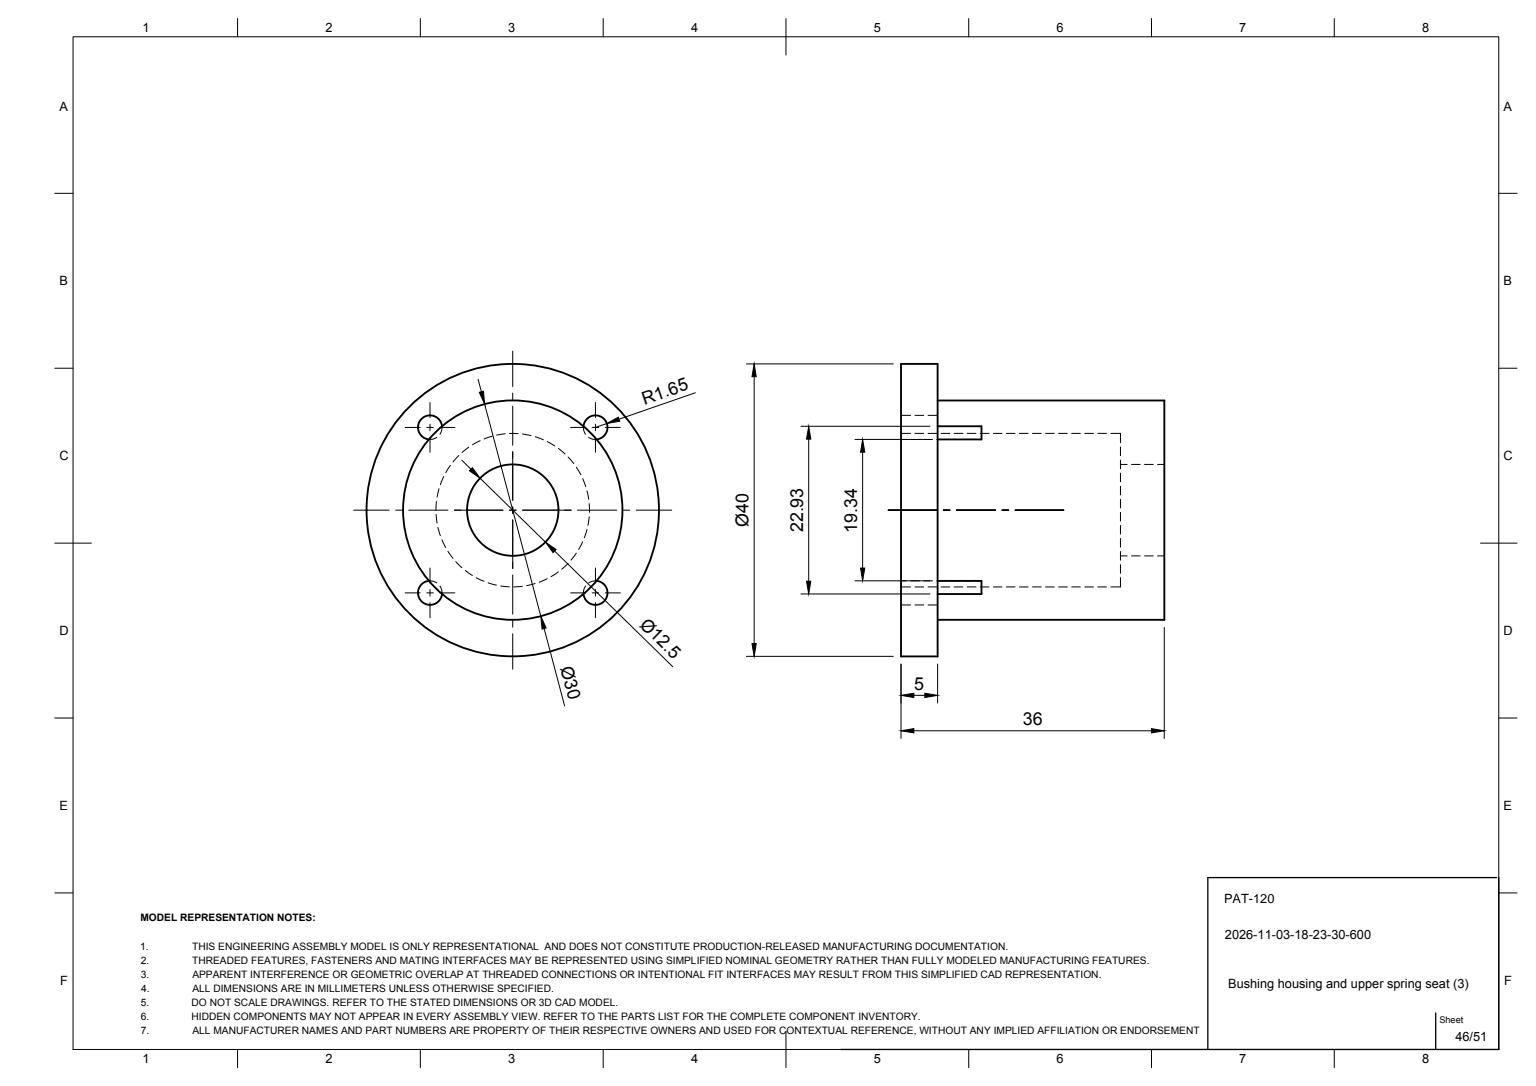
ISO-10303-21;
HEADER;
/* Generated by software containing ST-Developer
 * from STEP Tools, Inc. (www.steptools.com) 
 */

FILE_DESCRIPTION(
/* description */ ('Vibration shaker table dummy'),
/* implementation_level */ '2;1');

FILE_NAME(
/* name */ 'Bushing housing and upper spring seat (3).step',
/* time_stamp */ '2026-10-27T10:55:14-07:00',
/* author */ (''),
/* organization */ (''),
/* preprocessor_version */ 'ST-DEVELOPER v20.2',
/* originating_system */ 'Autodesk Translation Framework v15.17.0.0',
/* authorisation */ '');

FILE_SCHEMA (('AUTOMOTIVE_DESIGN { 1 0 10303 214 3 1 1 }'));
ENDSEC;

DATA;
#10=MECHANICAL_DESIGN_GEOMETRIC_PRESENTATION_REPRESENTATION('',(#727),#22394);
#635=SHAPE_REPRESENTATION_RELATIONSHIP('SRR','None',#22682,#681);
#681=ADVANCED_BREP_SHAPE_REPRESENTATION('',(#771),#22388);
#727=STYLED_ITEM('',(#22961),#771);
#771=MANIFOLD_SOLID_BREP('Body1',#9247);
#1031=FACE_BOUND('',#2537,.T.);
#1032=FACE_BOUND('',#2539,.T.);
#1033=FACE_BOUND('',#2543,.T.);
#1034=FACE_BOUND('',#2544,.T.);
#1035=FACE_BOUND('',#2545,.T.);
#1036=FACE_BOUND('',#2546,.T.);
#1037=FACE_BOUND('',#2547,.T.);
#1038=FACE_BOUND('',#2549,.T.);
#1302=PLANE('',#10665);
#1303=PLANE('',#10672);
#1304=PLANE('',#10679);
#1305=PLANE('',#10686);
#1306=PLANE('',#10703);
#1307=PLANE('',#10705);
#1308=PLANE('',#10711);
#1309=PLANE('',#10712);
#1772=FACE_OUTER_BOUND('',#2526,.T.);
#1773=FACE_OUTER_BOUND('',#2527,.T.);
#1774=FACE_OUTER_BOUND('',#2528,.T.);
#1775=FACE_OUTER_BOUND('',#2529,.T.);
#1776=FACE_OUTER_BOUND('',#2530,.T.);
#1777=FACE_OUTER_BOUND('',#2531,.T.);
#1778=FACE_OUTER_BOUND('',#2532,.T.);
#1779=FACE_OUTER_BOUND('',#2533,.T.);
#1780=FACE_OUTER_BOUND('',#2534,.T.);
#1781=FACE_OUTER_BOUND('',#2535,.T.);
#1782=FACE_OUTER_BOUND('',#2536,.T.);
#1783=FACE_OUTER_BOUND('',#2538,.T.);
#1784=FACE_OUTER_BOUND('',#2540,.T.);
#1785=FACE_OUTER_BOUND('',#2541,.T.);
#1786=FACE_OUTER_BOUND('',#2542,.T.);
#1787=FACE_OUTER_BOUND('',#2548,.T.);
#2526=EDGE_LOOP('',(#8214,#8215));
#2527=EDGE_LOOP('',(#8216,#8217,#8218,#8219,#8220,#8221,#8222,#8223));
#2528=EDGE_LOOP('',(#8224,#8225));
#2529=EDGE_LOOP('',(#8226,#8227,#8228,#8229,#8230,#8231,#8232,#8233));
#2530=EDGE_LOOP('',(#8234,#8235,#8236));
#2531=EDGE_LOOP('',(#8237,#8238,#8239,#8240,#8241,#8242,#8243,#8244));
#2532=EDGE_LOOP('',(#8245,#8246,#8247));
#2533=EDGE_LOOP('',(#8248,#8249,#8250,#8251,#8252,#8253,#8254,#8255));
#2534=EDGE_LOOP('',(#8256,#8257,#8258,#8259,#8260,#8261,#8262,#8263,#8264,
#8265,#8266,#8267,#8268,#8269,#8270,#8271,#8272,#8273,#8274,#8275));
#2535=EDGE_LOOP('',(#8276,#8277,#8278,#8279));
#2536=EDGE_LOOP('',(#8280));
#2537=EDGE_LOOP('',(#8281));
#2538=EDGE_LOOP('',(#8282));
#2539=EDGE_LOOP('',(#8283,#8284,#8285,#8286,#8287,#8288,#8289,#8290,#8291,
#8292,#8293));
#2540=EDGE_LOOP('',(#8294,#8295,#8296,#8297));
#2541=EDGE_LOOP('',(#8298,#8299,#8300,#8301));
#2542=EDGE_LOOP('',(#8302));
#2543=EDGE_LOOP('',(#8303));
#2544=EDGE_LOOP('',(#8304));
#2545=EDGE_LOOP('',(#8305));
#2546=EDGE_LOOP('',(#8306));
#2547=EDGE_LOOP('',(#8307));
#2548=EDGE_LOOP('',(#8308));
#2549=EDGE_LOOP('',(#8309));
#3169=LINE('',#21847,#3788);
#3170=LINE('',#21851,#3789);
#3171=LINE('',#21855,#3790);
#3172=LINE('',#21863,#3791);
#3173=LINE('',#21867,#3792);
#3174=LINE('',#21871,#3793);
#3175=LINE('',#21881,#3794);
#3176=LINE('',#21884,#3795);
#3177=LINE('',#21886,#3796);
#3178=LINE('',#21897,#3797);
#3179=LINE('',#21900,#3798);
#3180=LINE('',#21902,#3799);
#3181=LINE('',#21908,#3800);
#3182=LINE('',#21918,#3801);
#3183=LINE('',#21929,#3802);
#3184=LINE('',#21932,#3803);
#3788=VECTOR('',#13315,1.);
#3789=VECTOR('',#13318,0.165);
#3790=VECTOR('',#13323,1.);
#3791=VECTOR('',#13332,1.);
#3792=VECTOR('',#13335,0.165);
#3793=VECTOR('',#13340,1.);
#3794=VECTOR('',#13351,1.);
#3795=VECTOR('',#13354,1.);
#3796=VECTOR('',#13355,0.165);
#3797=VECTOR('',#13368,1.);
#3798=VECTOR('',#13371,1.);
#3799=VECTOR('',#13372,0.165);
#3800=VECTOR('',#13379,1.5);
#3801=VECTOR('',#13394,1.05);
#3802=VECTOR('',#13409,2.);
#3803=VECTOR('',#13412,0.625);
#4293=CIRCLE('',#10666,1.5);
#4294=CIRCLE('',#10667,0.165);
#4295=CIRCLE('',#10669,0.165);
#4296=CIRCLE('',#10670,0.165);
#4297=CIRCLE('',#10671,0.165);
#4298=CIRCLE('',#10673,1.5);
#4299=CIRCLE('',#10674,0.165);
#4300=CIRCLE('',#10676,0.165);
#4301=CIRCLE('',#10677,0.165);
#4302=CIRCLE('',#10678,0.165);
#4303=CIRCLE('',#10680,1.5);
#4304=CIRCLE('',#10681,0.165);
#4305=CIRCLE('',#10682,0.165);
#4306=CIRCLE('',#10684,0.165);
#4307=CIRCLE('',#10685,0.165);
#4308=CIRCLE('',#10687,1.5);
#4309=CIRCLE('',#10688,0.165);
#4310=CIRCLE('',#10689,0.165);
#4311=CIRCLE('',#10691,0.165);
#4312=CIRCLE('',#10692,0.165);
#4313=CIRCLE('',#10694,1.5);
#4314=CIRCLE('',#10695,1.5);
#4315=CIRCLE('',#10696,1.5);
#4316=CIRCLE('',#10697,1.5);
#4317=CIRCLE('',#10698,1.5);
#4318=CIRCLE('',#10699,1.5);
#4319=CIRCLE('',#10701,1.05);
#4320=CIRCLE('',#10702,1.05);
#4321=CIRCLE('',#10704,0.625);
#4322=CIRCLE('',#10706,2.);
#4323=CIRCLE('',#10708,2.);
#4324=CIRCLE('',#10710,0.625);
#5020=VERTEX_POINT('',#21841);
#5021=VERTEX_POINT('',#21842);
#5022=VERTEX_POINT('',#21846);
#5023=VERTEX_POINT('',#21848);
#5024=VERTEX_POINT('',#21850);
#5025=VERTEX_POINT('',#21853);
#5026=VERTEX_POINT('',#21857);
#5027=VERTEX_POINT('',#21858);
#5028=VERTEX_POINT('',#21862);
#5029=VERTEX_POINT('',#21864);
#5030=VERTEX_POINT('',#21866);
#5031=VERTEX_POINT('',#21869);
#5032=VERTEX_POINT('',#21873);
#5033=VERTEX_POINT('',#21874);
#5034=VERTEX_POINT('',#21876);
#5035=VERTEX_POINT('',#21880);
#5036=VERTEX_POINT('',#21882);
#5037=VERTEX_POINT('',#21885);
#5038=VERTEX_POINT('',#21889);
#5039=VERTEX_POINT('',#21890);
#5040=VERTEX_POINT('',#21892);
#5041=VERTEX_POINT('',#21896);
#5042=VERTEX_POINT('',#21898);
#5043=VERTEX_POINT('',#21901);
#5044=VERTEX_POINT('',#21905);
#5045=VERTEX_POINT('',#21907);
#5046=VERTEX_POINT('',#21915);
#5047=VERTEX_POINT('',#21917);
#5048=VERTEX_POINT('',#21921);
#5049=VERTEX_POINT('',#21924);
#5050=VERTEX_POINT('',#21927);
#5051=VERTEX_POINT('',#21931);
#6100=EDGE_CURVE('',#5020,#5021,#4293,.T.);
#6101=EDGE_CURVE('',#5020,#5021,#4294,.T.);
#6102=EDGE_CURVE('',#5022,#5020,#3169,.T.);
#6103=EDGE_CURVE('',#5023,#5022,#4295,.T.);
#6104=EDGE_CURVE('',#5023,#5024,#3170,.T.);
#6105=EDGE_CURVE('',#5024,#5024,#4296,.T.);
#6106=EDGE_CURVE('',#5025,#5023,#4297,.T.);
#6107=EDGE_CURVE('',#5021,#5025,#3171,.T.);
#6108=EDGE_CURVE('',#5026,#5027,#4298,.T.);
#6109=EDGE_CURVE('',#5026,#5027,#4299,.T.);
#6110=EDGE_CURVE('',#5028,#5026,#3172,.T.);
#6111=EDGE_CURVE('',#5029,#5028,#4300,.T.);
#6112=EDGE_CURVE('',#5029,#5030,#3173,.T.);
#6113=EDGE_CURVE('',#5030,#5030,#4301,.T.);
#6114=EDGE_CURVE('',#5031,#5029,#4302,.T.);
#6115=EDGE_CURVE('',#5027,#5031,#3174,.T.);
#6116=EDGE_CURVE('',#5032,#5033,#4303,.T.);
#6117=EDGE_CURVE('',#5032,#5034,#4304,.T.);
#6118=EDGE_CURVE('',#5034,#5033,#4305,.T.);
#6119=EDGE_CURVE('',#5035,#5032,#3175,.T.);
#6120=EDGE_CURVE('',#5036,#5035,#4306,.T.);
#6121=EDGE_CURVE('',#5033,#5036,#3176,.T.);
#6122=EDGE_CURVE('',#5034,#5037,#3177,.T.);
#6123=EDGE_CURVE('',#5037,#5037,#4307,.T.);
#6124=EDGE_CURVE('',#5038,#5039,#4308,.T.);
#6125=EDGE_CURVE('',#5038,#5040,#4309,.T.);
#6126=EDGE_CURVE('',#5040,#5039,#4310,.T.);
#6127=EDGE_CURVE('',#5041,#5038,#3178,.T.);
#6128=EDGE_CURVE('',#5042,#5041,#4311,.T.);
#6129=EDGE_CURVE('',#5039,#5042,#3179,.T.);
#6130=EDGE_CURVE('',#5040,#5043,#3180,.T.);
#6131=EDGE_CURVE('',#5043,#5043,#4312,.T.);
#6132=EDGE_CURVE('',#5025,#5044,#4313,.T.);
#6133=EDGE_CURVE('',#5044,#5045,#3181,.T.);
#6134=EDGE_CURVE('',#5045,#5045,#4314,.T.);
#6135=EDGE_CURVE('',#5044,#5028,#4315,.T.);
#6136=EDGE_CURVE('',#5031,#5035,#4316,.T.);
#6137=EDGE_CURVE('',#5036,#5041,#4317,.T.);
#6138=EDGE_CURVE('',#5042,#5022,#4318,.T.);
#6139=EDGE_CURVE('',#5046,#5046,#4319,.T.);
#6140=EDGE_CURVE('',#5046,#5047,#3182,.T.);
#6141=EDGE_CURVE('',#5047,#5047,#4320,.T.);
#6142=EDGE_CURVE('',#5048,#5048,#4321,.T.);
#6143=EDGE_CURVE('',#5049,#5049,#4322,.T.);
#6144=EDGE_CURVE('',#5050,#5050,#4323,.T.);
#6145=EDGE_CURVE('',#5050,#5049,#3183,.T.);
#6146=EDGE_CURVE('',#5048,#5051,#3184,.T.);
#6147=EDGE_CURVE('',#5051,#5051,#4324,.T.);
#8214=ORIENTED_EDGE('',*,*,#6100,.F.);
#8215=ORIENTED_EDGE('',*,*,#6101,.T.);
#8216=ORIENTED_EDGE('',*,*,#6102,.F.);
#8217=ORIENTED_EDGE('',*,*,#6103,.F.);
#8218=ORIENTED_EDGE('',*,*,#6104,.T.);
#8219=ORIENTED_EDGE('',*,*,#6105,.F.);
#8220=ORIENTED_EDGE('',*,*,#6104,.F.);
#8221=ORIENTED_EDGE('',*,*,#6106,.F.);
#8222=ORIENTED_EDGE('',*,*,#6107,.F.);
#8223=ORIENTED_EDGE('',*,*,#6101,.F.);
#8224=ORIENTED_EDGE('',*,*,#6108,.F.);
#8225=ORIENTED_EDGE('',*,*,#6109,.T.);
#8226=ORIENTED_EDGE('',*,*,#6110,.F.);
#8227=ORIENTED_EDGE('',*,*,#6111,.F.);
#8228=ORIENTED_EDGE('',*,*,#6112,.T.);
#8229=ORIENTED_EDGE('',*,*,#6113,.F.);
#8230=ORIENTED_EDGE('',*,*,#6112,.F.);
#8231=ORIENTED_EDGE('',*,*,#6114,.F.);
#8232=ORIENTED_EDGE('',*,*,#6115,.F.);
#8233=ORIENTED_EDGE('',*,*,#6109,.F.);
#8234=ORIENTED_EDGE('',*,*,#6116,.F.);
#8235=ORIENTED_EDGE('',*,*,#6117,.T.);
#8236=ORIENTED_EDGE('',*,*,#6118,.T.);
#8237=ORIENTED_EDGE('',*,*,#6119,.F.);
#8238=ORIENTED_EDGE('',*,*,#6120,.F.);
#8239=ORIENTED_EDGE('',*,*,#6121,.F.);
#8240=ORIENTED_EDGE('',*,*,#6118,.F.);
#8241=ORIENTED_EDGE('',*,*,#6122,.T.);
#8242=ORIENTED_EDGE('',*,*,#6123,.F.);
#8243=ORIENTED_EDGE('',*,*,#6122,.F.);
#8244=ORIENTED_EDGE('',*,*,#6117,.F.);
#8245=ORIENTED_EDGE('',*,*,#6124,.F.);
#8246=ORIENTED_EDGE('',*,*,#6125,.T.);
#8247=ORIENTED_EDGE('',*,*,#6126,.T.);
#8248=ORIENTED_EDGE('',*,*,#6127,.F.);
#8249=ORIENTED_EDGE('',*,*,#6128,.F.);
#8250=ORIENTED_EDGE('',*,*,#6129,.F.);
#8251=ORIENTED_EDGE('',*,*,#6126,.F.);
#8252=ORIENTED_EDGE('',*,*,#6130,.T.);
#8253=ORIENTED_EDGE('',*,*,#6131,.F.);
#8254=ORIENTED_EDGE('',*,*,#6130,.F.);
#8255=ORIENTED_EDGE('',*,*,#6125,.F.);
#8256=ORIENTED_EDGE('',*,*,#6102,.T.);
#8257=ORIENTED_EDGE('',*,*,#6100,.T.);
#8258=ORIENTED_EDGE('',*,*,#6107,.T.);
#8259=ORIENTED_EDGE('',*,*,#6132,.T.);
#8260=ORIENTED_EDGE('',*,*,#6133,.T.);
#8261=ORIENTED_EDGE('',*,*,#6134,.T.);
#8262=ORIENTED_EDGE('',*,*,#6133,.F.);
#8263=ORIENTED_EDGE('',*,*,#6135,.T.);
#8264=ORIENTED_EDGE('',*,*,#6110,.T.);
#8265=ORIENTED_EDGE('',*,*,#6108,.T.);
#8266=ORIENTED_EDGE('',*,*,#6115,.T.);
#8267=ORIENTED_EDGE('',*,*,#6136,.T.);
#8268=ORIENTED_EDGE('',*,*,#6119,.T.);
#8269=ORIENTED_EDGE('',*,*,#6116,.T.);
#8270=ORIENTED_EDGE('',*,*,#6121,.T.);
#8271=ORIENTED_EDGE('',*,*,#6137,.T.);
#8272=ORIENTED_EDGE('',*,*,#6127,.T.);
#8273=ORIENTED_EDGE('',*,*,#6124,.T.);
#8274=ORIENTED_EDGE('',*,*,#6129,.T.);
#8275=ORIENTED_EDGE('',*,*,#6138,.T.);
#8276=ORIENTED_EDGE('',*,*,#6139,.F.);
#8277=ORIENTED_EDGE('',*,*,#6140,.T.);
#8278=ORIENTED_EDGE('',*,*,#6141,.F.);
#8279=ORIENTED_EDGE('',*,*,#6140,.F.);
#8280=ORIENTED_EDGE('',*,*,#6139,.T.);
#8281=ORIENTED_EDGE('',*,*,#6142,.F.);
#8282=ORIENTED_EDGE('',*,*,#6143,.F.);
#8283=ORIENTED_EDGE('',*,*,#6106,.T.);
#8284=ORIENTED_EDGE('',*,*,#6103,.T.);
#8285=ORIENTED_EDGE('',*,*,#6138,.F.);
#8286=ORIENTED_EDGE('',*,*,#6128,.T.);
#8287=ORIENTED_EDGE('',*,*,#6137,.F.);
#8288=ORIENTED_EDGE('',*,*,#6120,.T.);
#8289=ORIENTED_EDGE('',*,*,#6136,.F.);
#8290=ORIENTED_EDGE('',*,*,#6114,.T.);
#8291=ORIENTED_EDGE('',*,*,#6111,.T.);
#8292=ORIENTED_EDGE('',*,*,#6135,.F.);
#8293=ORIENTED_EDGE('',*,*,#6132,.F.);
#8294=ORIENTED_EDGE('',*,*,#6144,.F.);
#8295=ORIENTED_EDGE('',*,*,#6145,.T.);
#8296=ORIENTED_EDGE('',*,*,#6143,.T.);
#8297=ORIENTED_EDGE('',*,*,#6145,.F.);
#8298=ORIENTED_EDGE('',*,*,#6142,.T.);
#8299=ORIENTED_EDGE('',*,*,#6146,.T.);
#8300=ORIENTED_EDGE('',*,*,#6147,.T.);
#8301=ORIENTED_EDGE('',*,*,#6146,.F.);
#8302=ORIENTED_EDGE('',*,*,#6144,.T.);
#8303=ORIENTED_EDGE('',*,*,#6141,.T.);
#8304=ORIENTED_EDGE('',*,*,#6131,.T.);
#8305=ORIENTED_EDGE('',*,*,#6123,.T.);
#8306=ORIENTED_EDGE('',*,*,#6113,.T.);
#8307=ORIENTED_EDGE('',*,*,#6105,.T.);
#8308=ORIENTED_EDGE('',*,*,#6134,.F.);
#8309=ORIENTED_EDGE('',*,*,#6147,.F.);
#8682=CYLINDRICAL_SURFACE('',#10668,0.165);
#8683=CYLINDRICAL_SURFACE('',#10675,0.165);
#8684=CYLINDRICAL_SURFACE('',#10683,0.165);
#8685=CYLINDRICAL_SURFACE('',#10690,0.165);
#8686=CYLINDRICAL_SURFACE('',#10693,1.5);
#8687=CYLINDRICAL_SURFACE('',#10700,1.05);
#8688=CYLINDRICAL_SURFACE('',#10707,2.);
#8689=CYLINDRICAL_SURFACE('',#10709,0.625);
#9137=ADVANCED_FACE('',(#1772),#1302,.T.);
#9138=ADVANCED_FACE('',(#1773),#8682,.F.);
#9139=ADVANCED_FACE('',(#1774),#1303,.T.);
#9140=ADVANCED_FACE('',(#1775),#8683,.F.);
#9141=ADVANCED_FACE('',(#1776),#1304,.T.);
#9142=ADVANCED_FACE('',(#1777),#8684,.F.);
#9143=ADVANCED_FACE('',(#1778),#1305,.T.);
#9144=ADVANCED_FACE('',(#1779),#8685,.F.);
#9145=ADVANCED_FACE('',(#1780),#8686,.T.);
#9146=ADVANCED_FACE('',(#1781),#8687,.F.);
#9147=ADVANCED_FACE('',(#1782,#1031),#1306,.T.);
#9148=ADVANCED_FACE('',(#1783,#1032),#1307,.F.);
#9149=ADVANCED_FACE('',(#1784),#8688,.T.);
#9150=ADVANCED_FACE('',(#1785),#8689,.F.);
#9151=ADVANCED_FACE('',(#1786,#1033,#1034,#1035,#1036,#1037),#1308,.T.);
#9152=ADVANCED_FACE('',(#1787,#1038),#1309,.F.);
#9247=CLOSED_SHELL('',(#9137,#9138,#9139,#9140,#9141,#9142,#9143,#9144,
#9145,#9146,#9147,#9148,#9149,#9150,#9151,#9152));
#10664=AXIS2_PLACEMENT_3D('',#21839,#13305,#13306);
#10665=AXIS2_PLACEMENT_3D('',#21840,#13307,#13308);
#10666=AXIS2_PLACEMENT_3D('',#21843,#13309,#13310);
#10667=AXIS2_PLACEMENT_3D('',#21844,#13311,#13312);
#10668=AXIS2_PLACEMENT_3D('',#21845,#13313,#13314);
#10669=AXIS2_PLACEMENT_3D('',#21849,#13316,#13317);
#10670=AXIS2_PLACEMENT_3D('',#21852,#13319,#13320);
#10671=AXIS2_PLACEMENT_3D('',#21854,#13321,#13322);
#10672=AXIS2_PLACEMENT_3D('',#21856,#13324,#13325);
#10673=AXIS2_PLACEMENT_3D('',#21859,#13326,#13327);
#10674=AXIS2_PLACEMENT_3D('',#21860,#13328,#13329);
#10675=AXIS2_PLACEMENT_3D('',#21861,#13330,#13331);
#10676=AXIS2_PLACEMENT_3D('',#21865,#13333,#13334);
#10677=AXIS2_PLACEMENT_3D('',#21868,#13336,#13337);
#10678=AXIS2_PLACEMENT_3D('',#21870,#13338,#13339);
#10679=AXIS2_PLACEMENT_3D('',#21872,#13341,#13342);
#10680=AXIS2_PLACEMENT_3D('',#21875,#13343,#13344);
#10681=AXIS2_PLACEMENT_3D('',#21877,#13345,#13346);
#10682=AXIS2_PLACEMENT_3D('',#21878,#13347,#13348);
#10683=AXIS2_PLACEMENT_3D('',#21879,#13349,#13350);
#10684=AXIS2_PLACEMENT_3D('',#21883,#13352,#13353);
#10685=AXIS2_PLACEMENT_3D('',#21887,#13356,#13357);
#10686=AXIS2_PLACEMENT_3D('',#21888,#13358,#13359);
#10687=AXIS2_PLACEMENT_3D('',#21891,#13360,#13361);
#10688=AXIS2_PLACEMENT_3D('',#21893,#13362,#13363);
#10689=AXIS2_PLACEMENT_3D('',#21894,#13364,#13365);
#10690=AXIS2_PLACEMENT_3D('',#21895,#13366,#13367);
#10691=AXIS2_PLACEMENT_3D('',#21899,#13369,#13370);
#10692=AXIS2_PLACEMENT_3D('',#21903,#13373,#13374);
#10693=AXIS2_PLACEMENT_3D('',#21904,#13375,#13376);
#10694=AXIS2_PLACEMENT_3D('',#21906,#13377,#13378);
#10695=AXIS2_PLACEMENT_3D('',#21909,#13380,#13381);
#10696=AXIS2_PLACEMENT_3D('',#21910,#13382,#13383);
#10697=AXIS2_PLACEMENT_3D('',#21911,#13384,#13385);
#10698=AXIS2_PLACEMENT_3D('',#21912,#13386,#13387);
#10699=AXIS2_PLACEMENT_3D('',#21913,#13388,#13389);
#10700=AXIS2_PLACEMENT_3D('',#21914,#13390,#13391);
#10701=AXIS2_PLACEMENT_3D('',#21916,#13392,#13393);
#10702=AXIS2_PLACEMENT_3D('',#21919,#13395,#13396);
#10703=AXIS2_PLACEMENT_3D('',#21920,#13397,#13398);
#10704=AXIS2_PLACEMENT_3D('',#21922,#13399,#13400);
#10705=AXIS2_PLACEMENT_3D('',#21923,#13401,#13402);
#10706=AXIS2_PLACEMENT_3D('',#21925,#13403,#13404);
#10707=AXIS2_PLACEMENT_3D('',#21926,#13405,#13406);
#10708=AXIS2_PLACEMENT_3D('',#21928,#13407,#13408);
#10709=AXIS2_PLACEMENT_3D('',#21930,#13410,#13411);
#10710=AXIS2_PLACEMENT_3D('',#21933,#13413,#13414);
#10711=AXIS2_PLACEMENT_3D('',#21934,#13415,#13416);
#10712=AXIS2_PLACEMENT_3D('',#21935,#13417,#13418);
#13305=DIRECTION('axis',(0.,0.,1.));
#13306=DIRECTION('refdir',(1.,0.,0.));
#13307=DIRECTION('center_axis',(0.,0.,1.));
#13308=DIRECTION('ref_axis',(1.,0.,0.));
#13309=DIRECTION('center_axis',(0.,0.,-1.));
#13310=DIRECTION('ref_axis',(1.,0.,0.));
#13311=DIRECTION('center_axis',(0.,0.,1.));
#13312=DIRECTION('ref_axis',(1.,0.,0.));
#13313=DIRECTION('center_axis',(0.,0.,1.));
#13314=DIRECTION('ref_axis',(1.,0.,0.));
#13315=DIRECTION('',(0.,0.,-1.));
#13316=DIRECTION('center_axis',(0.,0.,1.));
#13317=DIRECTION('ref_axis',(1.,0.,0.));
#13318=DIRECTION('',(0.,0.,1.));
#13319=DIRECTION('center_axis',(0.,0.,-1.));
#13320=DIRECTION('ref_axis',(1.,0.,0.));
#13321=DIRECTION('center_axis',(0.,0.,1.));
#13322=DIRECTION('ref_axis',(1.,0.,0.));
#13323=DIRECTION('',(0.,0.,1.));
#13324=DIRECTION('center_axis',(0.,0.,1.));
#13325=DIRECTION('ref_axis',(1.,0.,0.));
#13326=DIRECTION('center_axis',(0.,0.,-1.));
#13327=DIRECTION('ref_axis',(1.,0.,0.));
#13328=DIRECTION('center_axis',(0.,0.,1.));
#13329=DIRECTION('ref_axis',(1.,0.,0.));
#13330=DIRECTION('center_axis',(0.,0.,1.));
#13331=DIRECTION('ref_axis',(1.,0.,0.));
#13332=DIRECTION('',(0.,0.,-1.));
#13333=DIRECTION('center_axis',(0.,0.,1.));
#13334=DIRECTION('ref_axis',(1.,0.,0.));
#13335=DIRECTION('',(0.,0.,1.));
#13336=DIRECTION('center_axis',(0.,0.,-1.));
#13337=DIRECTION('ref_axis',(1.,0.,0.));
#13338=DIRECTION('center_axis',(0.,0.,1.));
#13339=DIRECTION('ref_axis',(1.,0.,0.));
#13340=DIRECTION('',(0.,0.,1.));
#13341=DIRECTION('center_axis',(0.,0.,1.));
#13342=DIRECTION('ref_axis',(1.,0.,0.));
#13343=DIRECTION('center_axis',(0.,0.,-1.));
#13344=DIRECTION('ref_axis',(1.,0.,0.));
#13345=DIRECTION('center_axis',(0.,0.,1.));
#13346=DIRECTION('ref_axis',(1.,0.,0.));
#13347=DIRECTION('center_axis',(0.,0.,1.));
#13348=DIRECTION('ref_axis',(1.,0.,0.));
#13349=DIRECTION('center_axis',(0.,0.,1.));
#13350=DIRECTION('ref_axis',(1.,0.,0.));
#13351=DIRECTION('',(0.,0.,-1.));
#13352=DIRECTION('center_axis',(0.,0.,1.));
#13353=DIRECTION('ref_axis',(1.,0.,0.));
#13354=DIRECTION('',(0.,0.,1.));
#13355=DIRECTION('',(0.,0.,1.));
#13356=DIRECTION('center_axis',(0.,0.,-1.));
#13357=DIRECTION('ref_axis',(1.,0.,0.));
#13358=DIRECTION('center_axis',(0.,0.,1.));
#13359=DIRECTION('ref_axis',(1.,0.,0.));
#13360=DIRECTION('center_axis',(0.,0.,-1.));
#13361=DIRECTION('ref_axis',(1.,0.,0.));
#13362=DIRECTION('center_axis',(0.,0.,1.));
#13363=DIRECTION('ref_axis',(1.,0.,0.));
#13364=DIRECTION('center_axis',(0.,0.,1.));
#13365=DIRECTION('ref_axis',(1.,0.,0.));
#13366=DIRECTION('center_axis',(0.,0.,1.));
#13367=DIRECTION('ref_axis',(1.,0.,0.));
#13368=DIRECTION('',(0.,0.,-1.));
#13369=DIRECTION('center_axis',(0.,0.,1.));
#13370=DIRECTION('ref_axis',(1.,0.,0.));
#13371=DIRECTION('',(0.,0.,1.));
#13372=DIRECTION('',(0.,0.,1.));
#13373=DIRECTION('center_axis',(0.,0.,-1.));
#13374=DIRECTION('ref_axis',(1.,0.,0.));
#13375=DIRECTION('center_axis',(0.,0.,1.));
#13376=DIRECTION('ref_axis',(1.,0.,0.));
#13377=DIRECTION('center_axis',(0.,0.,-1.));
#13378=DIRECTION('ref_axis',(1.,0.,0.));
#13379=DIRECTION('',(0.,0.,-1.));
#13380=DIRECTION('center_axis',(0.,0.,1.));
#13381=DIRECTION('ref_axis',(1.,0.,0.));
#13382=DIRECTION('center_axis',(0.,0.,-1.));
#13383=DIRECTION('ref_axis',(1.,0.,0.));
#13384=DIRECTION('center_axis',(0.,0.,-1.));
#13385=DIRECTION('ref_axis',(1.,0.,0.));
#13386=DIRECTION('center_axis',(0.,0.,-1.));
#13387=DIRECTION('ref_axis',(1.,0.,0.));
#13388=DIRECTION('center_axis',(0.,0.,-1.));
#13389=DIRECTION('ref_axis',(1.,0.,0.));
#13390=DIRECTION('center_axis',(0.,0.,1.));
#13391=DIRECTION('ref_axis',(1.,0.,0.));
#13392=DIRECTION('center_axis',(0.,0.,1.));
#13393=DIRECTION('ref_axis',(1.,0.,0.));
#13394=DIRECTION('',(0.,0.,1.));
#13395=DIRECTION('center_axis',(0.,0.,-1.));
#13396=DIRECTION('ref_axis',(1.,0.,0.));
#13397=DIRECTION('center_axis',(0.,0.,1.));
#13398=DIRECTION('ref_axis',(1.,0.,0.));
#13399=DIRECTION('center_axis',(0.,0.,1.));
#13400=DIRECTION('ref_axis',(1.,0.,0.));
#13401=DIRECTION('center_axis',(0.,0.,1.));
#13402=DIRECTION('ref_axis',(1.,0.,0.));
#13403=DIRECTION('center_axis',(0.,0.,1.));
#13404=DIRECTION('ref_axis',(1.,0.,0.));
#13405=DIRECTION('center_axis',(0.,0.,1.));
#13406=DIRECTION('ref_axis',(1.,0.,0.));
#13407=DIRECTION('center_axis',(0.,0.,1.));
#13408=DIRECTION('ref_axis',(1.,0.,0.));
#13409=DIRECTION('',(0.,0.,-1.));
#13410=DIRECTION('center_axis',(0.,0.,1.));
#13411=DIRECTION('ref_axis',(1.,0.,0.));
#13412=DIRECTION('',(0.,0.,-1.));
#13413=DIRECTION('center_axis',(0.,0.,-1.));
#13414=DIRECTION('ref_axis',(1.,0.,0.));
#13415=DIRECTION('center_axis',(0.,0.,1.));
#13416=DIRECTION('ref_axis',(1.,0.,0.));
#13417=DIRECTION('center_axis',(0.,0.,1.));
#13418=DIRECTION('ref_axis',(1.,0.,0.));
#21839=CARTESIAN_POINT('',(0.,0.,0.));
#21840=CARTESIAN_POINT('Origin',(4.86862915010152,2.86862915010152,14.));
#21841=CARTESIAN_POINT('',(5.03292205834015,2.85337004454142,14.));
#21842=CARTESIAN_POINT('',(4.85337004454142,3.03292205834015,14.));
#21843=CARTESIAN_POINT('Origin',(6.,4.,14.));
#21844=CARTESIAN_POINT('Origin',(4.86862915010152,2.86862915010152,14.));
#21845=CARTESIAN_POINT('Origin',(4.86862915010152,2.86862915010152,14.));
#21846=CARTESIAN_POINT('',(5.03292205834015,2.85337004454142,14.6));
#21847=CARTESIAN_POINT('',(5.03292205834015,2.85337004454142,14.));
#21848=CARTESIAN_POINT('',(4.70362915010152,2.86862915010152,14.6));
#21849=CARTESIAN_POINT('Origin',(4.86862915010152,2.86862915010152,14.6));
#21850=CARTESIAN_POINT('',(4.70362915010152,2.86862915010152,15.1));
#21851=CARTESIAN_POINT('',(4.70362915010152,2.86862915010152,14.));
#21852=CARTESIAN_POINT('Origin',(4.86862915010152,2.86862915010152,15.1));
#21853=CARTESIAN_POINT('',(4.85337004454142,3.03292205834015,14.6));
#21854=CARTESIAN_POINT('Origin',(4.86862915010152,2.86862915010152,14.6));
#21855=CARTESIAN_POINT('',(4.85337004454142,3.03292205834015,14.));
#21856=CARTESIAN_POINT('Origin',(4.86862915010152,5.13137084989848,14.));
#21857=CARTESIAN_POINT('',(4.85337004454142,4.96707794165985,14.));
#21858=CARTESIAN_POINT('',(5.03292205834015,5.14662995545858,14.));
#21859=CARTESIAN_POINT('Origin',(6.,4.,14.));
#21860=CARTESIAN_POINT('Origin',(4.86862915010152,5.13137084989848,14.));
#21861=CARTESIAN_POINT('Origin',(4.86862915010152,5.13137084989848,14.));
#21862=CARTESIAN_POINT('',(4.85337004454142,4.96707794165985,14.6));
#21863=CARTESIAN_POINT('',(4.85337004454142,4.96707794165985,14.));
#21864=CARTESIAN_POINT('',(4.70362915010152,5.13137084989848,14.6));
#21865=CARTESIAN_POINT('Origin',(4.86862915010152,5.13137084989848,14.6));
#21866=CARTESIAN_POINT('',(4.70362915010152,5.13137084989848,15.1));
#21867=CARTESIAN_POINT('',(4.70362915010152,5.13137084989848,14.));
#21868=CARTESIAN_POINT('Origin',(4.86862915010152,5.13137084989848,15.1));
#21869=CARTESIAN_POINT('',(5.03292205834015,5.14662995545858,14.6));
#21870=CARTESIAN_POINT('Origin',(4.86862915010152,5.13137084989848,14.6));
#21871=CARTESIAN_POINT('',(5.03292205834015,5.14662995545858,14.));
#21872=CARTESIAN_POINT('Origin',(7.13137084989848,5.13137084989848,14.));
#21873=CARTESIAN_POINT('',(6.96707794165985,5.14662995545858,14.));
#21874=CARTESIAN_POINT('',(7.14662995545858,4.96707794165985,14.));
#21875=CARTESIAN_POINT('Origin',(6.,4.,14.));
#21876=CARTESIAN_POINT('',(6.96637084989848,5.13137084989848,14.));
#21877=CARTESIAN_POINT('Origin',(7.13137084989848,5.13137084989848,14.));
#21878=CARTESIAN_POINT('Origin',(7.13137084989848,5.13137084989848,14.));
#21879=CARTESIAN_POINT('Origin',(7.13137084989848,5.13137084989848,14.));
#21880=CARTESIAN_POINT('',(6.96707794165985,5.14662995545858,14.6));
#21881=CARTESIAN_POINT('',(6.96707794165985,5.14662995545858,14.));
#21882=CARTESIAN_POINT('',(7.14662995545858,4.96707794165985,14.6));
#21883=CARTESIAN_POINT('Origin',(7.13137084989848,5.13137084989848,14.6));
#21884=CARTESIAN_POINT('',(7.14662995545858,4.96707794165985,14.));
#21885=CARTESIAN_POINT('',(6.96637084989848,5.13137084989848,15.1));
#21886=CARTESIAN_POINT('',(6.96637084989848,5.13137084989848,14.));
#21887=CARTESIAN_POINT('Origin',(7.13137084989848,5.13137084989848,15.1));
#21888=CARTESIAN_POINT('Origin',(7.13137084989848,2.86862915010152,14.));
#21889=CARTESIAN_POINT('',(7.14662995545858,3.03292205834015,14.));
#21890=CARTESIAN_POINT('',(6.96707794165985,2.85337004454142,14.));
#21891=CARTESIAN_POINT('Origin',(6.,4.,14.));
#21892=CARTESIAN_POINT('',(6.96637084989848,2.86862915010152,14.));
#21893=CARTESIAN_POINT('Origin',(7.13137084989848,2.86862915010152,14.));
#21894=CARTESIAN_POINT('Origin',(7.13137084989848,2.86862915010152,14.));
#21895=CARTESIAN_POINT('Origin',(7.13137084989848,2.86862915010152,14.));
#21896=CARTESIAN_POINT('',(7.14662995545858,3.03292205834015,14.6));
#21897=CARTESIAN_POINT('',(7.14662995545858,3.03292205834015,14.));
#21898=CARTESIAN_POINT('',(6.96707794165985,2.85337004454142,14.6));
#21899=CARTESIAN_POINT('Origin',(7.13137084989848,2.86862915010152,14.6));
#21900=CARTESIAN_POINT('',(6.96707794165985,2.85337004454142,14.));
#21901=CARTESIAN_POINT('',(6.96637084989848,2.86862915010152,15.1));
#21902=CARTESIAN_POINT('',(6.96637084989848,2.86862915010152,14.));
#21903=CARTESIAN_POINT('Origin',(7.13137084989848,2.86862915010152,15.1));
#21904=CARTESIAN_POINT('Origin',(6.,4.,11.5));
#21905=CARTESIAN_POINT('',(4.5,4.,14.6));
#21906=CARTESIAN_POINT('Origin',(6.,4.,14.6));
#21907=CARTESIAN_POINT('',(4.5,4.,11.5));
#21908=CARTESIAN_POINT('',(4.5,4.,11.5));
#21909=CARTESIAN_POINT('Origin',(6.,4.,11.5));
#21910=CARTESIAN_POINT('Origin',(6.,4.,14.6));
#21911=CARTESIAN_POINT('Origin',(6.,4.,14.6));
#21912=CARTESIAN_POINT('Origin',(6.,4.,14.6));
#21913=CARTESIAN_POINT('Origin',(6.,4.,14.6));
#21914=CARTESIAN_POINT('Origin',(6.,4.,12.1));
#21915=CARTESIAN_POINT('',(4.95,4.,12.1));
#21916=CARTESIAN_POINT('Origin',(6.,4.,12.1));
#21917=CARTESIAN_POINT('',(4.95,4.,15.1));
#21918=CARTESIAN_POINT('',(4.95,4.,12.1));
#21919=CARTESIAN_POINT('Origin',(6.,4.,15.1));
#21920=CARTESIAN_POINT('Origin',(6.,4.,12.1));
#21921=CARTESIAN_POINT('',(5.375,4.,12.1));
#21922=CARTESIAN_POINT('Origin',(6.,4.,12.1));
#21923=CARTESIAN_POINT('Origin',(6.,4.,14.6));
#21924=CARTESIAN_POINT('',(4.,4.,14.6));
#21925=CARTESIAN_POINT('Origin',(6.,4.,14.6));
#21926=CARTESIAN_POINT('Origin',(6.,4.,14.6));
#21927=CARTESIAN_POINT('',(4.,4.,15.1));
#21928=CARTESIAN_POINT('Origin',(6.,4.,15.1));
#21929=CARTESIAN_POINT('',(4.,4.,14.6));
#21930=CARTESIAN_POINT('Origin',(6.,4.,11.5));
#21931=CARTESIAN_POINT('',(5.375,4.,11.5));
#21932=CARTESIAN_POINT('',(5.375,4.,11.5));
#21933=CARTESIAN_POINT('Origin',(6.,4.,11.5));
#21934=CARTESIAN_POINT('Origin',(6.,4.,15.1));
#21935=CARTESIAN_POINT('Origin',(6.,4.,11.5));
#22337=UNCERTAINTY_MEASURE_WITH_UNIT(LENGTH_MEASURE(0.001),#22395,
'DISTANCE_ACCURACY_VALUE',
'Maximum model space distance between geometric entities at asserted c
onnectivities');
#22343=UNCERTAINTY_MEASURE_WITH_UNIT(LENGTH_MEASURE(0.001),#22395,
'DISTANCE_ACCURACY_VALUE',
'Maximum model space distance between geometric entities at asserted c
onnectivities');
#22388=(
GEOMETRIC_REPRESENTATION_CONTEXT(3)
GLOBAL_UNCERTAINTY_ASSIGNED_CONTEXT((#22337))
GLOBAL_UNIT_ASSIGNED_CONTEXT((#22395,#22397,#22398))
REPRESENTATION_CONTEXT('','3D')
);
#22394=(
GEOMETRIC_REPRESENTATION_CONTEXT(3)
GLOBAL_UNCERTAINTY_ASSIGNED_CONTEXT((#22343))
GLOBAL_UNIT_ASSIGNED_CONTEXT((#22395,#22397,#22398))
REPRESENTATION_CONTEXT('','3D')
);
#22395=(
LENGTH_UNIT()
NAMED_UNIT(*)
SI_UNIT(.CENTI.,.METRE.)
);
#22397=(
NAMED_UNIT(*)
PLANE_ANGLE_UNIT()
SI_UNIT($,.RADIAN.)
);
#22398=(
NAMED_UNIT(*)
SI_UNIT($,.STERADIAN.)
SOLID_ANGLE_UNIT()
);
#22443=SHAPE_DEFINITION_REPRESENTATION(#22493,#22682);
#22493=PRODUCT_DEFINITION_SHAPE('',$,#22733);
#22682=SHAPE_REPRESENTATION('',(#10664),#22388);
#22688=PRODUCT_DEFINITION_CONTEXT('part definition',#22840,'design');
#22733=PRODUCT_DEFINITION('Bushing housing and upper spring seat (3)',
'Bushing housing and upper spring seat (3)',#22783,#22688);
#22783=PRODUCT_DEFINITION_FORMATION('',$,#22886);
#22840=APPLICATION_CONTEXT(
'Core Data for Automotive Mechanical Design Process');
#22841=PRODUCT_CONTEXT('part definition',#22840,'mechanical');
#22886=PRODUCT('Bushing housing and upper spring seat (3)',
'Bushing housing and upper spring seat (3)',
'Bushing housing and upper spring seat (3)',(#22841));
#22955=COLOUR_RGB('Grey',0.48,0.52,0.57);
#22956=FILL_AREA_STYLE_COLOUR('',#22955);
#22957=FILL_AREA_STYLE('',(#22956));
#22958=SURFACE_STYLE_FILL_AREA(#22957);
#22959=SURFACE_SIDE_STYLE('',(#22958));
#22960=SURFACE_STYLE_USAGE(.BOTH.,#22959);
#22961=PRESENTATION_STYLE_ASSIGNMENT((#22960));
ENDSEC;
END-ISO-10303-21;
